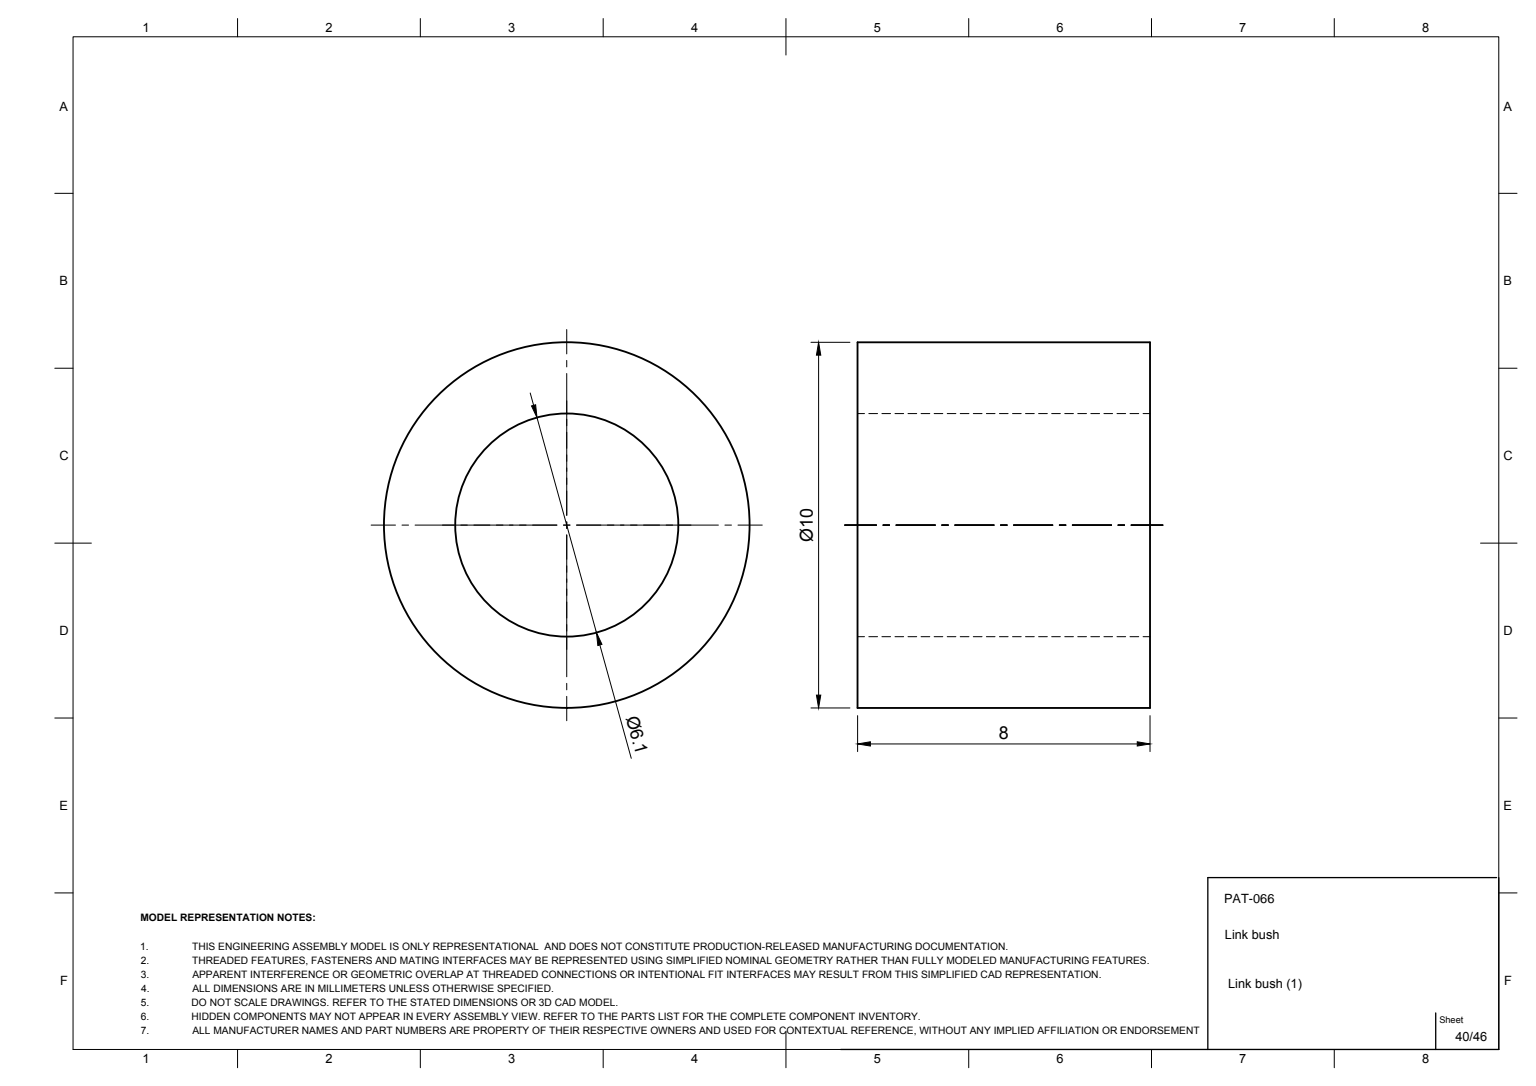
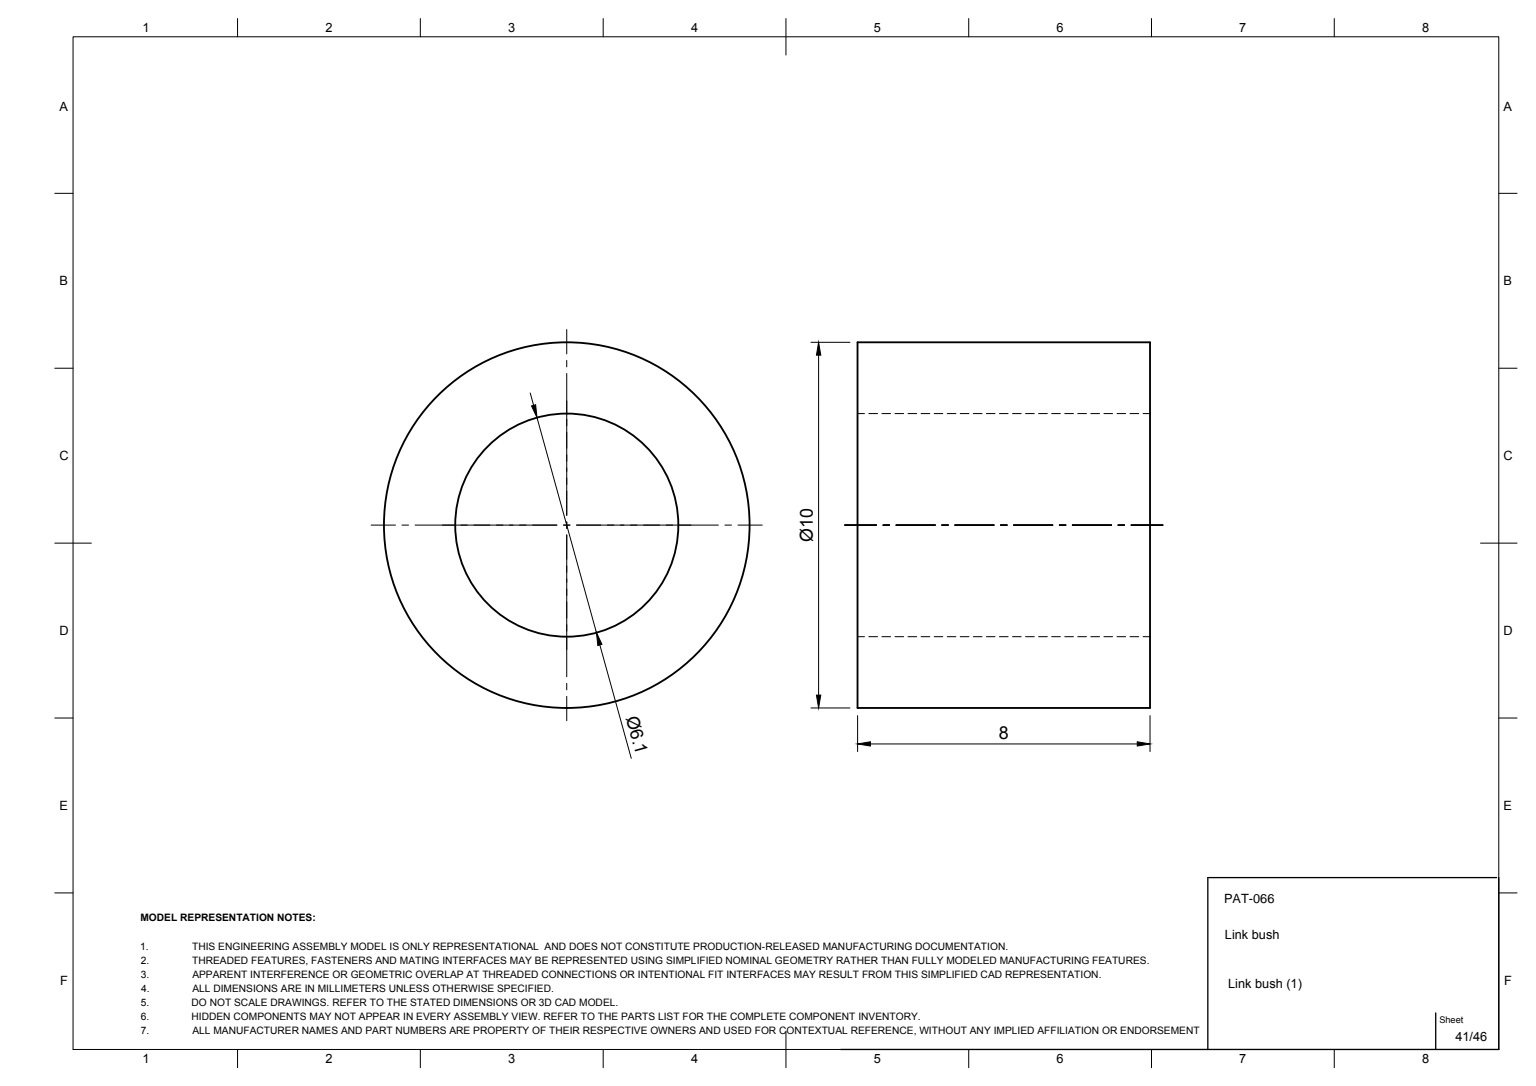
ISO-10303-21;
HEADER;
/* Generated by software containing ST-Developer
 * from STEP Tools, Inc. (www.steptools.com) 
 */

FILE_DESCRIPTION(
/* description */ ('Lever-operated bar clamp (toggle)'),
/* implementation_level */ '2;1');

FILE_NAME(
/* name */ 'Link bush.step',
/* time_stamp */ '2026-10-28T03:25:02-07:00',
/* author */ (''),
/* organization */ (''),
/* preprocessor_version */ 'ST-DEVELOPER v20.2',
/* originating_system */ 'Autodesk Translation Framework v15.17.0.0',
/* authorisation */ '');

FILE_SCHEMA (('AUTOMOTIVE_DESIGN { 1 0 10303 214 3 1 1 }'));
ENDSEC;

DATA;
#10=MECHANICAL_DESIGN_GEOMETRIC_PRESENTATION_REPRESENTATION('',(#450),#12413);
#366=SHAPE_REPRESENTATION_RELATIONSHIP('SRR','None',#12609,#404);
#404=ADVANCED_BREP_SHAPE_REPRESENTATION('',(#493),#12406);
#450=STYLED_ITEM('',(#12883),#493);
#493=MANIFOLD_SOLID_BREP('Body1',#6613);
#640=FACE_BOUND('',#1791,.T.);
#641=FACE_BOUND('',#1793,.T.);
#851=PLANE('',#7798);
#852=PLANE('',#7799);
#1242=FACE_OUTER_BOUND('',#1788,.T.);
#1243=FACE_OUTER_BOUND('',#1789,.T.);
#1244=FACE_OUTER_BOUND('',#1790,.T.);
#1245=FACE_OUTER_BOUND('',#1792,.T.);
#1788=EDGE_LOOP('',(#5829,#5830,#5831,#5832));
#1789=EDGE_LOOP('',(#5833,#5834,#5835,#5836));
#1790=EDGE_LOOP('',(#5837));
#1791=EDGE_LOOP('',(#5838));
#1792=EDGE_LOOP('',(#5839));
#1793=EDGE_LOOP('',(#5840));
#2225=LINE('',#12070,#2666);
#2226=LINE('',#12076,#2667);
#2666=VECTOR('',#9778,0.305);
#2667=VECTOR('',#9785,0.5);
#3041=CIRCLE('',#7793,0.305);
#3042=CIRCLE('',#7794,0.305);
#3043=CIRCLE('',#7796,0.5);
#3044=CIRCLE('',#7797,0.5);
#3548=VERTEX_POINT('',#12067);
#3549=VERTEX_POINT('',#12069);
#3550=VERTEX_POINT('',#12073);
#3551=VERTEX_POINT('',#12075);
#4319=EDGE_CURVE('',#3548,#3548,#3041,.T.);
#4320=EDGE_CURVE('',#3548,#3549,#2225,.T.);
#4321=EDGE_CURVE('',#3549,#3549,#3042,.T.);
#4322=EDGE_CURVE('',#3550,#3550,#3043,.T.);
#4323=EDGE_CURVE('',#3550,#3551,#2226,.T.);
#4324=EDGE_CURVE('',#3551,#3551,#3044,.T.);
#5829=ORIENTED_EDGE('',*,*,#4319,.F.);
#5830=ORIENTED_EDGE('',*,*,#4320,.T.);
#5831=ORIENTED_EDGE('',*,*,#4321,.T.);
#5832=ORIENTED_EDGE('',*,*,#4320,.F.);
#5833=ORIENTED_EDGE('',*,*,#4322,.F.);
#5834=ORIENTED_EDGE('',*,*,#4323,.T.);
#5835=ORIENTED_EDGE('',*,*,#4324,.T.);
#5836=ORIENTED_EDGE('',*,*,#4323,.F.);
#5837=ORIENTED_EDGE('',*,*,#4322,.T.);
#5838=ORIENTED_EDGE('',*,*,#4319,.T.);
#5839=ORIENTED_EDGE('',*,*,#4324,.F.);
#5840=ORIENTED_EDGE('',*,*,#4321,.F.);
#6150=CYLINDRICAL_SURFACE('',#7792,0.305);
#6151=CYLINDRICAL_SURFACE('',#7795,0.5);
#6517=ADVANCED_FACE('',(#1242),#6150,.F.);
#6518=ADVANCED_FACE('',(#1243),#6151,.T.);
#6519=ADVANCED_FACE('',(#1244,#640),#851,.T.);
#6520=ADVANCED_FACE('',(#1245,#641),#852,.F.);
#6613=CLOSED_SHELL('',(#6517,#6518,#6519,#6520));
#7791=AXIS2_PLACEMENT_3D('',#12065,#9772,#9773);
#7792=AXIS2_PLACEMENT_3D('',#12066,#9774,#9775);
#7793=AXIS2_PLACEMENT_3D('',#12068,#9776,#9777);
#7794=AXIS2_PLACEMENT_3D('',#12071,#9779,#9780);
#7795=AXIS2_PLACEMENT_3D('',#12072,#9781,#9782);
#7796=AXIS2_PLACEMENT_3D('',#12074,#9783,#9784);
#7797=AXIS2_PLACEMENT_3D('',#12077,#9786,#9787);
#7798=AXIS2_PLACEMENT_3D('',#12078,#9788,#9789);
#7799=AXIS2_PLACEMENT_3D('',#12079,#9790,#9791);
#9772=DIRECTION('axis',(0.,0.,1.));
#9773=DIRECTION('refdir',(1.,0.,0.));
#9774=DIRECTION('center_axis',(0.,1.,0.));
#9775=DIRECTION('ref_axis',(1.,0.,0.));
#9776=DIRECTION('center_axis',(0.,-1.,0.));
#9777=DIRECTION('ref_axis',(1.,0.,0.));
#9778=DIRECTION('',(0.,-1.,0.));
#9779=DIRECTION('center_axis',(0.,-1.,0.));
#9780=DIRECTION('ref_axis',(1.,0.,0.));
#9781=DIRECTION('center_axis',(0.,1.,0.));
#9782=DIRECTION('ref_axis',(1.,0.,0.));
#9783=DIRECTION('center_axis',(0.,1.,0.));
#9784=DIRECTION('ref_axis',(1.,0.,0.));
#9785=DIRECTION('',(0.,-1.,0.));
#9786=DIRECTION('center_axis',(0.,1.,0.));
#9787=DIRECTION('ref_axis',(1.,0.,0.));
#9788=DIRECTION('center_axis',(0.,1.,0.));
#9789=DIRECTION('ref_axis',(1.,0.,0.));
#9790=DIRECTION('center_axis',(0.,1.,0.));
#9791=DIRECTION('ref_axis',(1.,0.,0.));
#12065=CARTESIAN_POINT('',(0.,0.,0.));
#12066=CARTESIAN_POINT('Origin',(-2.82632109303527,-5.5,8.79263101785268));
#12067=CARTESIAN_POINT('',(-3.13132109303527,-4.7,8.79263101785268));
#12068=CARTESIAN_POINT('Origin',(-2.82632109303527,-4.7,8.79263101785268));
#12069=CARTESIAN_POINT('',(-3.13132109303527,-5.5,8.79263101785268));
#12070=CARTESIAN_POINT('',(-3.13132109303527,-5.5,8.79263101785268));
#12071=CARTESIAN_POINT('Origin',(-2.82632109303527,-5.5,8.79263101785268));
#12072=CARTESIAN_POINT('Origin',(-2.82632109303527,-5.5,8.79263101785268));
#12073=CARTESIAN_POINT('',(-3.32632109303527,-4.7,8.79263101785268));
#12074=CARTESIAN_POINT('Origin',(-2.82632109303527,-4.7,8.79263101785268));
#12075=CARTESIAN_POINT('',(-3.32632109303527,-5.5,8.79263101785268));
#12076=CARTESIAN_POINT('',(-3.32632109303527,-5.5,8.79263101785268));
#12077=CARTESIAN_POINT('Origin',(-2.82632109303527,-5.5,8.79263101785268));
#12078=CARTESIAN_POINT('Origin',(-2.82632109303527,-4.7,8.79263101785268));
#12079=CARTESIAN_POINT('Origin',(-2.82632109303527,-5.5,8.79263101785268));
#12360=UNCERTAINTY_MEASURE_WITH_UNIT(LENGTH_MEASURE(0.001),#12414,
'DISTANCE_ACCURACY_VALUE',
'Maximum model space distance between geometric entities at asserted c
onnectivities');
#12367=UNCERTAINTY_MEASURE_WITH_UNIT(LENGTH_MEASURE(0.001),#12414,
'DISTANCE_ACCURACY_VALUE',
'Maximum model space distance between geometric entities at asserted c
onnectivities');
#12406=(
GEOMETRIC_REPRESENTATION_CONTEXT(3)
GLOBAL_UNCERTAINTY_ASSIGNED_CONTEXT((#12360))
GLOBAL_UNIT_ASSIGNED_CONTEXT((#12414,#12416,#12417))
REPRESENTATION_CONTEXT('','3D')
);
#12413=(
GEOMETRIC_REPRESENTATION_CONTEXT(3)
GLOBAL_UNCERTAINTY_ASSIGNED_CONTEXT((#12367))
GLOBAL_UNIT_ASSIGNED_CONTEXT((#12414,#12416,#12417))
REPRESENTATION_CONTEXT('','3D')
);
#12414=(
LENGTH_UNIT()
NAMED_UNIT(*)
SI_UNIT(.CENTI.,.METRE.)
);
#12416=(
NAMED_UNIT(*)
PLANE_ANGLE_UNIT()
SI_UNIT($,.RADIAN.)
);
#12417=(
NAMED_UNIT(*)
SI_UNIT($,.STERADIAN.)
SOLID_ANGLE_UNIT()
);
#12456=SHAPE_DEFINITION_REPRESENTATION(#12553,#12609);
#12553=PRODUCT_DEFINITION_SHAPE('',$,#12655);
#12609=SHAPE_REPRESENTATION('',(#7791),#12406);
#12616=PRODUCT_DEFINITION_CONTEXT('part definition',#12753,'design');
#12655=PRODUCT_DEFINITION('Link bush','Link bush',#12700,#12616);
#12700=PRODUCT_DEFINITION_FORMATION('',$,#12793);
#12753=APPLICATION_CONTEXT(
'Core Data for Automotive Mechanical Design Process');
#12754=PRODUCT_CONTEXT('part definition',#12753,'mechanical');
#12793=PRODUCT('Link bush','Link bush','Link bush',(#12754));
#12877=COLOUR_RGB('Off White',0.89,0.88,0.83);
#12878=FILL_AREA_STYLE_COLOUR('',#12877);
#12879=FILL_AREA_STYLE('',(#12878));
#12880=SURFACE_STYLE_FILL_AREA(#12879);
#12881=SURFACE_SIDE_STYLE('',(#12880));
#12882=SURFACE_STYLE_USAGE(.BOTH.,#12881);
#12883=PRESENTATION_STYLE_ASSIGNMENT((#12882));
ENDSEC;
END-ISO-10303-21;
